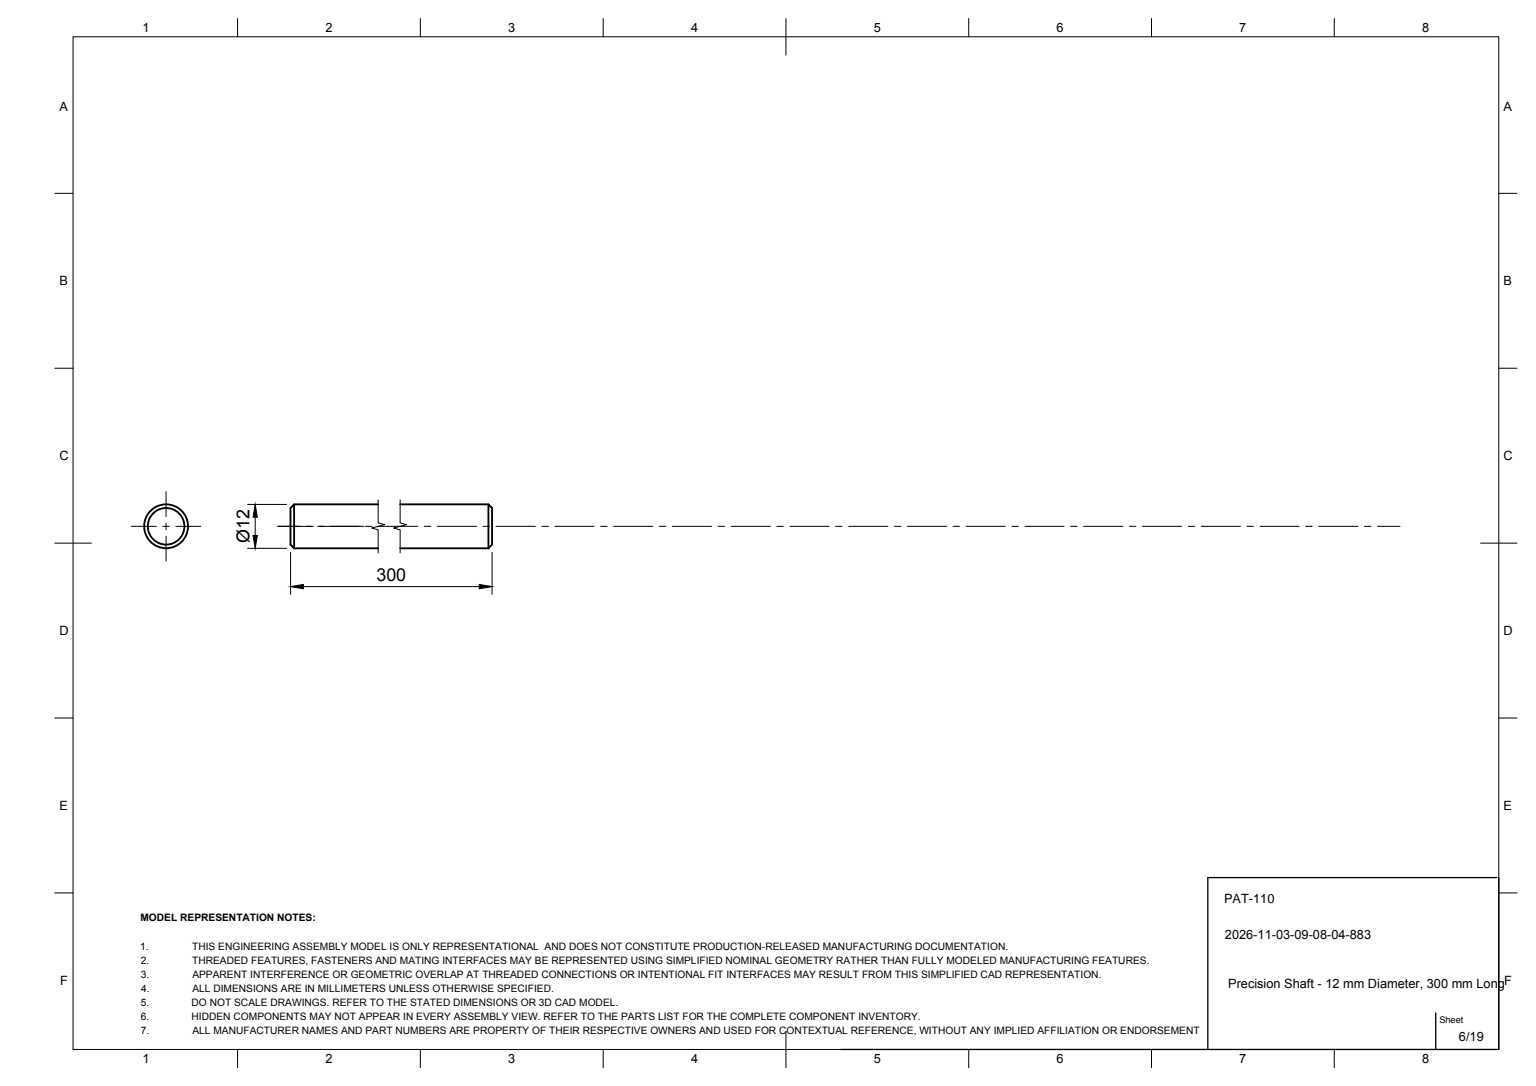
ISO-10303-21;
HEADER;
/* Generated by software containing ST-Developer
 * from STEP Tools, Inc. (www.steptools.com) 
 */

FILE_DESCRIPTION(
/* description */ ('Twin-shaft manual slide'),
/* implementation_level */ '2;1');

FILE_NAME(
/* name */ 'Precision Shaft - 12 mm Diameter, 300 mm Long.step',
/* time_stamp */ '2026-10-27T18:38:08-07:00',
/* author */ (''),
/* organization */ (''),
/* preprocessor_version */ 'ST-DEVELOPER v20.2',
/* originating_system */ 'Autodesk Translation Framework v15.17.0.0',
/* authorisation */ '');

FILE_SCHEMA (('AUTOMOTIVE_DESIGN { 1 0 10303 214 3 1 1 }'));
ENDSEC;

DATA;
#10=MECHANICAL_DESIGN_GEOMETRIC_PRESENTATION_REPRESENTATION('',(#277),#6463);
#227=CONICAL_SURFACE('',#3881,0.55,0.785398163397448);
#228=CONICAL_SURFACE('',#3887,0.55,0.785398163397441);
#245=SHAPE_REPRESENTATION_RELATIONSHIP('SRR','None',#6563,#261);
#261=ADVANCED_BREP_SHAPE_REPRESENTATION('',(#293),#6446);
#277=STYLED_ITEM('',(#6740),#293);
#293=MANIFOLD_SOLID_BREP('Body1',#3639);
#407=PLANE('',#3886);
#408=PLANE('',#3889);
#544=FACE_OUTER_BOUND('',#775,.T.);
#545=FACE_OUTER_BOUND('',#776,.T.);
#546=FACE_OUTER_BOUND('',#777,.T.);
#547=FACE_OUTER_BOUND('',#778,.T.);
#548=FACE_OUTER_BOUND('',#779,.T.);
#775=EDGE_LOOP('',(#2584,#2585,#2586,#2587));
#776=EDGE_LOOP('',(#2588,#2589,#2590,#2591));
#777=EDGE_LOOP('',(#2592));
#778=EDGE_LOOP('',(#2593,#2594,#2595,#2596));
#779=EDGE_LOOP('',(#2597));
#1061=LINE('',#5523,#1347);
#1062=LINE('',#5528,#1348);
#1063=LINE('',#5533,#1349);
#1347=VECTOR('',#4387,0.55);
#1348=VECTOR('',#4394,0.6);
#1349=VECTOR('',#4401,0.55);
#1633=CIRCLE('',#3882,0.6);
#1634=CIRCLE('',#3883,0.5);
#1635=CIRCLE('',#3885,0.6);
#1636=CIRCLE('',#3888,0.5);
#1794=VERTEX_POINT('',#5520);
#1795=VERTEX_POINT('',#5522);
#1796=VERTEX_POINT('',#5526);
#1797=VERTEX_POINT('',#5531);
#2097=EDGE_CURVE('',#1794,#1794,#1633,.T.);
#2098=EDGE_CURVE('',#1794,#1795,#1061,.T.);
#2099=EDGE_CURVE('',#1795,#1795,#1634,.T.);
#2100=EDGE_CURVE('',#1796,#1796,#1635,.T.);
#2101=EDGE_CURVE('',#1796,#1794,#1062,.T.);
#2102=EDGE_CURVE('',#1797,#1797,#1636,.T.);
#2103=EDGE_CURVE('',#1797,#1796,#1063,.T.);
#2584=ORIENTED_EDGE('',*,*,#2097,.T.);
#2585=ORIENTED_EDGE('',*,*,#2098,.T.);
#2586=ORIENTED_EDGE('',*,*,#2099,.T.);
#2587=ORIENTED_EDGE('',*,*,#2098,.F.);
#2588=ORIENTED_EDGE('',*,*,#2100,.F.);
#2589=ORIENTED_EDGE('',*,*,#2101,.T.);
#2590=ORIENTED_EDGE('',*,*,#2097,.F.);
#2591=ORIENTED_EDGE('',*,*,#2101,.F.);
#2592=ORIENTED_EDGE('',*,*,#2099,.F.);
#2593=ORIENTED_EDGE('',*,*,#2102,.T.);
#2594=ORIENTED_EDGE('',*,*,#2103,.T.);
#2595=ORIENTED_EDGE('',*,*,#2100,.T.);
#2596=ORIENTED_EDGE('',*,*,#2103,.F.);
#2597=ORIENTED_EDGE('',*,*,#2102,.F.);
#3378=CYLINDRICAL_SURFACE('',#3884,0.6);
#3449=ADVANCED_FACE('',(#544),#227,.T.);
#3450=ADVANCED_FACE('',(#545),#3378,.T.);
#3451=ADVANCED_FACE('',(#546),#407,.F.);
#3452=ADVANCED_FACE('',(#547),#228,.T.);
#3453=ADVANCED_FACE('',(#548),#408,.T.);
#3639=CLOSED_SHELL('',(#3449,#3450,#3451,#3452,#3453));
#3880=AXIS2_PLACEMENT_3D('',#5518,#4381,#4382);
#3881=AXIS2_PLACEMENT_3D('',#5519,#4383,#4384);
#3882=AXIS2_PLACEMENT_3D('',#5521,#4385,#4386);
#3883=AXIS2_PLACEMENT_3D('',#5524,#4388,#4389);
#3884=AXIS2_PLACEMENT_3D('',#5525,#4390,#4391);
#3885=AXIS2_PLACEMENT_3D('',#5527,#4392,#4393);
#3886=AXIS2_PLACEMENT_3D('',#5529,#4395,#4396);
#3887=AXIS2_PLACEMENT_3D('',#5530,#4397,#4398);
#3888=AXIS2_PLACEMENT_3D('',#5532,#4399,#4400);
#3889=AXIS2_PLACEMENT_3D('',#5534,#4402,#4403);
#4381=DIRECTION('axis',(0.,0.,1.));
#4382=DIRECTION('refdir',(1.,0.,0.));
#4383=DIRECTION('center_axis',(1.,0.,0.));
#4384=DIRECTION('ref_axis',(0.,0.,-1.));
#4385=DIRECTION('center_axis',(-1.,0.,0.));
#4386=DIRECTION('ref_axis',(0.,0.,-1.));
#4387=DIRECTION('',(-0.707106781186548,8.65956056235493E-17,-0.707106781186547));
#4388=DIRECTION('center_axis',(1.,0.,0.));
#4389=DIRECTION('ref_axis',(0.,0.,-1.));
#4390=DIRECTION('center_axis',(1.,0.,0.));
#4391=DIRECTION('ref_axis',(0.,0.,-1.));
#4392=DIRECTION('center_axis',(1.,0.,0.));
#4393=DIRECTION('ref_axis',(0.,0.,-1.));
#4394=DIRECTION('',(-1.,0.,0.));
#4395=DIRECTION('center_axis',(1.,0.,0.));
#4396=DIRECTION('ref_axis',(0.,0.,-1.));
#4397=DIRECTION('center_axis',(-1.,0.,0.));
#4398=DIRECTION('ref_axis',(0.,0.,-1.));
#4399=DIRECTION('center_axis',(-1.,0.,0.));
#4400=DIRECTION('ref_axis',(0.,0.,-1.));
#4401=DIRECTION('',(-0.707106781186553,-8.65956056235487E-17,0.707106781186542));
#4402=DIRECTION('center_axis',(1.,0.,0.));
#4403=DIRECTION('ref_axis',(0.,0.,-1.));
#5518=CARTESIAN_POINT('',(0.,0.,0.));
#5519=CARTESIAN_POINT('Origin',(0.05,0.,0.));
#5520=CARTESIAN_POINT('',(0.1,7.34788079488412E-17,0.6));
#5521=CARTESIAN_POINT('Origin',(0.1,0.,0.));
#5522=CARTESIAN_POINT('',(0.,-6.12323399573677E-17,0.5));
#5523=CARTESIAN_POINT('',(0.05,-6.73555739531044E-17,0.55));
#5524=CARTESIAN_POINT('Origin',(0.,0.,0.));
#5525=CARTESIAN_POINT('Origin',(0.,0.,0.));
#5526=CARTESIAN_POINT('',(29.9,-7.34788079488412E-17,0.6));
#5527=CARTESIAN_POINT('Origin',(29.9,0.,0.));
#5528=CARTESIAN_POINT('',(0.,-7.34788079488412E-17,0.6));
#5529=CARTESIAN_POINT('Origin',(0.,0.,0.));
#5530=CARTESIAN_POINT('Origin',(29.95,0.,0.));
#5531=CARTESIAN_POINT('',(30.,6.12323399573677E-17,0.5));
#5532=CARTESIAN_POINT('Origin',(30.,0.,0.));
#5533=CARTESIAN_POINT('',(29.95,-6.73555739531044E-17,0.55));
#5534=CARTESIAN_POINT('Origin',(30.,0.,0.));
#6425=UNCERTAINTY_MEASURE_WITH_UNIT(LENGTH_MEASURE(0.001),#6464,
'DISTANCE_ACCURACY_VALUE',
'Maximum model space distance between geometric entities at asserted c
onnectivities');
#6442=UNCERTAINTY_MEASURE_WITH_UNIT(LENGTH_MEASURE(0.001),#6464,
'DISTANCE_ACCURACY_VALUE',
'Maximum model space distance between geometric entities at asserted c
onnectivities');
#6446=(
GEOMETRIC_REPRESENTATION_CONTEXT(3)
GLOBAL_UNCERTAINTY_ASSIGNED_CONTEXT((#6425))
GLOBAL_UNIT_ASSIGNED_CONTEXT((#6464,#6466,#6467))
REPRESENTATION_CONTEXT('','3D')
);
#6463=(
GEOMETRIC_REPRESENTATION_CONTEXT(3)
GLOBAL_UNCERTAINTY_ASSIGNED_CONTEXT((#6442))
GLOBAL_UNIT_ASSIGNED_CONTEXT((#6464,#6466,#6467))
REPRESENTATION_CONTEXT('','3D')
);
#6464=(
LENGTH_UNIT()
NAMED_UNIT(*)
SI_UNIT(.CENTI.,.METRE.)
);
#6466=(
NAMED_UNIT(*)
PLANE_ANGLE_UNIT()
SI_UNIT($,.RADIAN.)
);
#6467=(
NAMED_UNIT(*)
SI_UNIT($,.STERADIAN.)
SOLID_ANGLE_UNIT()
);
#6471=SHAPE_DEFINITION_REPRESENTATION(#6491,#6563);
#6491=PRODUCT_DEFINITION_SHAPE('',$,#6584);
#6563=SHAPE_REPRESENTATION('',(#3880),#6446);
#6580=PRODUCT_DEFINITION_CONTEXT('part definition',#6642,'design');
#6584=PRODUCT_DEFINITION(
'Precision Shaft - 12 mm Diameter, 300 mm Long',
'Precision Shaft - 12 mm Diameter, 300 mm Long',#6604,#6580);
#6604=PRODUCT_DEFINITION_FORMATION('',$,#6647);
#6642=APPLICATION_CONTEXT(
'Core Data for Automotive Mechanical Design Process');
#6643=PRODUCT_CONTEXT('part definition',#6642,'mechanical');
#6647=PRODUCT('Precision Shaft - 12 mm Diameter, 300 mm Long',
'Precision Shaft - 12 mm Diameter, 300 mm Long',
'Precision Shaft - 12 mm Diameter, 300 mm Long',(#6643));
#6734=COLOUR_RGB('Grey',0.48,0.52,0.57);
#6735=FILL_AREA_STYLE_COLOUR('',#6734);
#6736=FILL_AREA_STYLE('',(#6735));
#6737=SURFACE_STYLE_FILL_AREA(#6736);
#6738=SURFACE_SIDE_STYLE('',(#6737));
#6739=SURFACE_STYLE_USAGE(.BOTH.,#6738);
#6740=PRESENTATION_STYLE_ASSIGNMENT((#6739));
ENDSEC;
END-ISO-10303-21;
